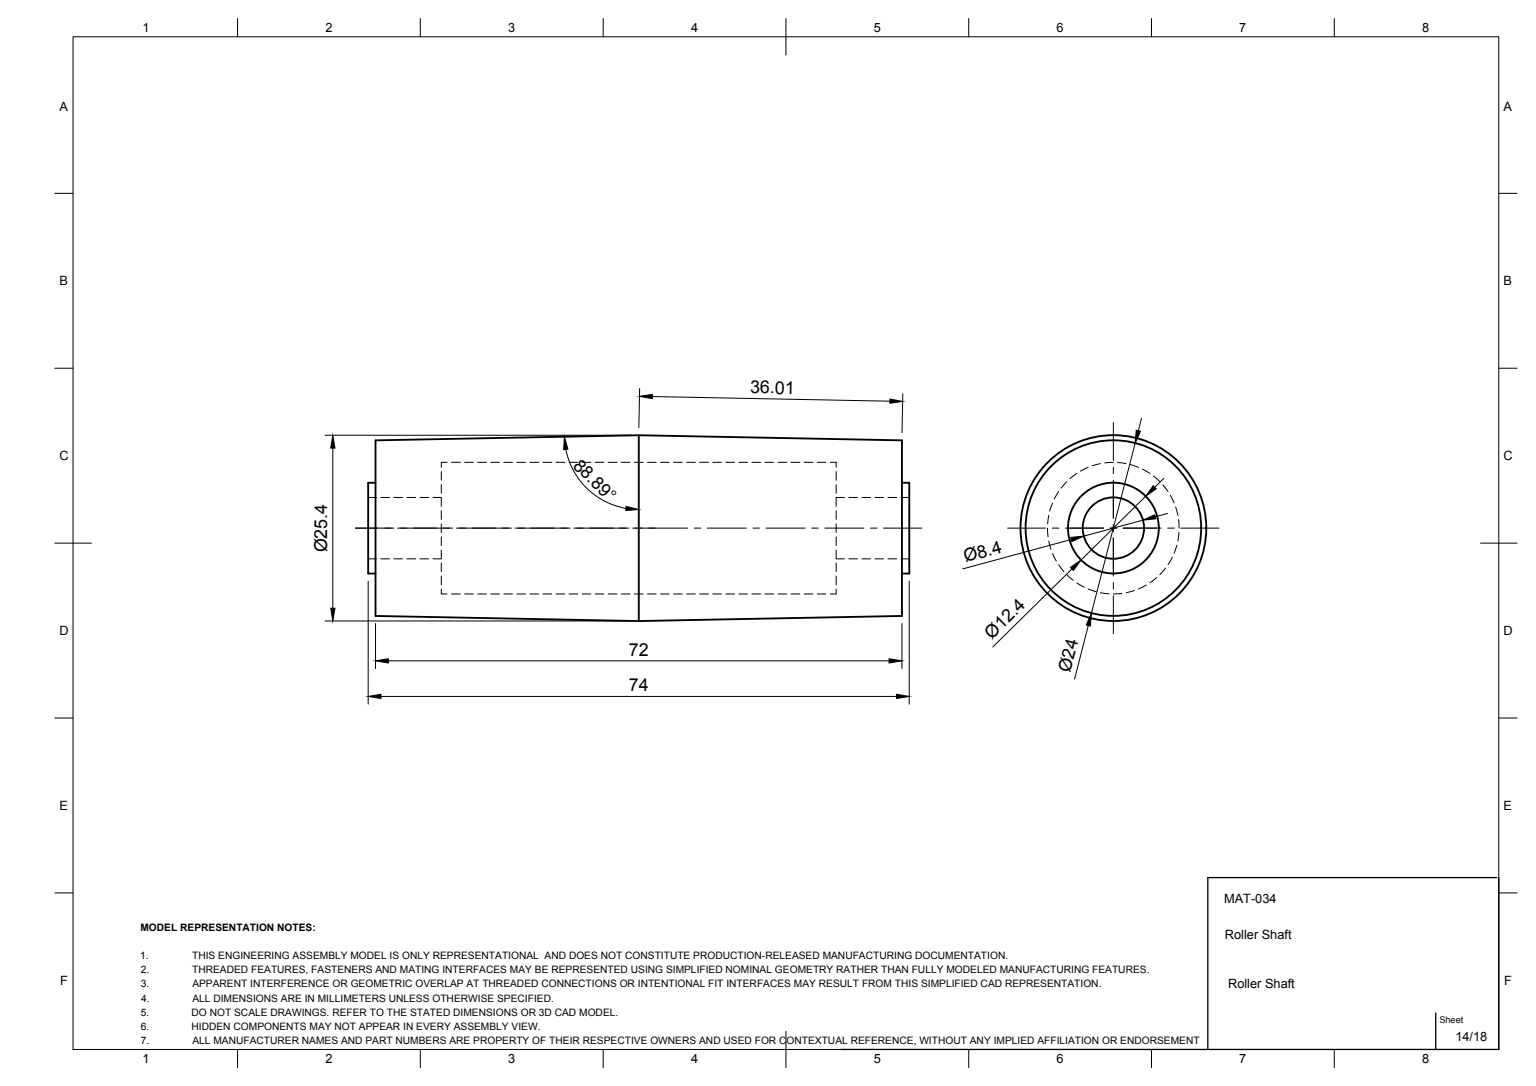
ISO-10303-21;
HEADER;
/* Generated by software containing ST-Developer
 * from STEP Tools, Inc. (www.steptools.com) 
 */

FILE_DESCRIPTION(
/* description */ ('STEP AP214'),
/* implementation_level */ '2;1');

FILE_NAME(
/* name */ 'Roller Shaft.step',
/* time_stamp */ '2026-11-14T09:24:36-08:00',
/* author */ (''),
/* organization */ (''),
/* preprocessor_version */ 'ST-DEVELOPER v20.2',
/* originating_system */ 'Autodesk Translation Framework v15.17.0.0',
/* authorisation */ '');

FILE_SCHEMA (('AUTOMOTIVE_DESIGN { 1 0 10303 214 3 1 1 }'));
ENDSEC;

DATA;
#10=MECHANICAL_DESIGN_GEOMETRIC_PRESENTATION_REPRESENTATION('',(#217),#18867);
#130=CONICAL_SURFACE('',#12139,12.7,0.0194419944400805);
#131=CONICAL_SURFACE('',#12143,12.7,0.0194419944400803);
#185=SHAPE_REPRESENTATION_RELATIONSHIP('SRR','None',#18949,#201);
#201=ADVANCED_BREP_SHAPE_REPRESENTATION('',(#241),#18865);
#217=STYLED_ITEM('',(#19027),#241);
#241=MANIFOLD_SOLID_BREP('Body1',#10972);
#367=FACE_BOUND('',#1981,.T.);
#368=FACE_BOUND('',#1983,.T.);
#369=FACE_BOUND('',#1985,.T.);
#370=FACE_BOUND('',#1987,.T.);
#371=FACE_BOUND('',#1989,.T.);
#372=FACE_BOUND('',#1991,.T.);
#711=PLANE('',#12157);
#712=PLANE('',#12158);
#713=PLANE('',#12159);
#714=PLANE('',#12160);
#715=PLANE('',#12161);
#716=PLANE('',#12162);
#1261=FACE_OUTER_BOUND('',#1973,.T.);
#1262=FACE_OUTER_BOUND('',#1974,.T.);
#1263=FACE_OUTER_BOUND('',#1975,.T.);
#1264=FACE_OUTER_BOUND('',#1976,.T.);
#1265=FACE_OUTER_BOUND('',#1977,.T.);
#1266=FACE_OUTER_BOUND('',#1978,.T.);
#1267=FACE_OUTER_BOUND('',#1979,.T.);
#1268=FACE_OUTER_BOUND('',#1980,.T.);
#1269=FACE_OUTER_BOUND('',#1982,.T.);
#1270=FACE_OUTER_BOUND('',#1984,.T.);
#1271=FACE_OUTER_BOUND('',#1986,.T.);
#1272=FACE_OUTER_BOUND('',#1988,.T.);
#1273=FACE_OUTER_BOUND('',#1990,.T.);
#1973=EDGE_LOOP('',(#9936,#9937,#9938,#9939));
#1974=EDGE_LOOP('',(#9940,#9941,#9942,#9943,#9944));
#1975=EDGE_LOOP('',(#9945,#9946,#9947,#9948,#9949));
#1976=EDGE_LOOP('',(#9950,#9951,#9952,#9953));
#1977=EDGE_LOOP('',(#9954,#9955,#9956,#9957));
#1978=EDGE_LOOP('',(#9958,#9959,#9960,#9961));
#1979=EDGE_LOOP('',(#9962,#9963,#9964,#9965));
#1980=EDGE_LOOP('',(#9966));
#1981=EDGE_LOOP('',(#9967));
#1982=EDGE_LOOP('',(#9968));
#1983=EDGE_LOOP('',(#9969));
#1984=EDGE_LOOP('',(#9970));
#1985=EDGE_LOOP('',(#9971));
#1986=EDGE_LOOP('',(#9972));
#1987=EDGE_LOOP('',(#9973));
#1988=EDGE_LOOP('',(#9974));
#1989=EDGE_LOOP('',(#9975));
#1990=EDGE_LOOP('',(#9976));
#1991=EDGE_LOOP('',(#9977));
#3032=LINE('',#18565,#4046);
#3033=LINE('',#18573,#4047);
#3034=LINE('',#18577,#4048);
#3035=LINE('',#18583,#4049);
#3036=LINE('',#18589,#4050);
#3037=LINE('',#18595,#4051);
#3038=LINE('',#18601,#4052);
#4046=VECTOR('',#15246,9.);
#4047=VECTOR('',#15255,12.7);
#4048=VECTOR('',#15260,12.7);
#4049=VECTOR('',#15267,6.2);
#4050=VECTOR('',#15274,6.2);
#4051=VECTOR('',#15281,4.2);
#4052=VECTOR('',#15288,4.2);
#4496=CIRCLE('',#12137,9.);
#4497=CIRCLE('',#12138,9.);
#4498=CIRCLE('',#12140,12.7);
#4499=CIRCLE('',#12141,12.7);
#4500=CIRCLE('',#12142,12.);
#4501=CIRCLE('',#12144,12.);
#4502=CIRCLE('',#12146,6.2);
#4503=CIRCLE('',#12147,6.2);
#4504=CIRCLE('',#12149,6.2);
#4505=CIRCLE('',#12150,6.2);
#4506=CIRCLE('',#12152,4.2);
#4507=CIRCLE('',#12153,4.2);
#4508=CIRCLE('',#12155,4.2);
#4509=CIRCLE('',#12156,4.2);
#5512=VERTEX_POINT('',#18562);
#5513=VERTEX_POINT('',#18564);
#5514=VERTEX_POINT('',#18568);
#5515=VERTEX_POINT('',#18569);
#5516=VERTEX_POINT('',#18572);
#5517=VERTEX_POINT('',#18576);
#5518=VERTEX_POINT('',#18580);
#5519=VERTEX_POINT('',#18582);
#5520=VERTEX_POINT('',#18586);
#5521=VERTEX_POINT('',#18588);
#5522=VERTEX_POINT('',#18592);
#5523=VERTEX_POINT('',#18594);
#5524=VERTEX_POINT('',#18598);
#5525=VERTEX_POINT('',#18600);
#7001=EDGE_CURVE('',#5512,#5512,#4496,.T.);
#7002=EDGE_CURVE('',#5512,#5513,#3032,.T.);
#7003=EDGE_CURVE('',#5513,#5513,#4497,.T.);
#7004=EDGE_CURVE('',#5514,#5515,#4498,.T.);
#7005=EDGE_CURVE('',#5515,#5514,#4499,.T.);
#7006=EDGE_CURVE('',#5515,#5516,#3033,.T.);
#7007=EDGE_CURVE('',#5516,#5516,#4500,.T.);
#7008=EDGE_CURVE('',#5514,#5517,#3034,.T.);
#7009=EDGE_CURVE('',#5517,#5517,#4501,.T.);
#7010=EDGE_CURVE('',#5518,#5518,#4502,.T.);
#7011=EDGE_CURVE('',#5518,#5519,#3035,.T.);
#7012=EDGE_CURVE('',#5519,#5519,#4503,.T.);
#7013=EDGE_CURVE('',#5520,#5520,#4504,.T.);
#7014=EDGE_CURVE('',#5520,#5521,#3036,.T.);
#7015=EDGE_CURVE('',#5521,#5521,#4505,.T.);
#7016=EDGE_CURVE('',#5522,#5522,#4506,.T.);
#7017=EDGE_CURVE('',#5522,#5523,#3037,.T.);
#7018=EDGE_CURVE('',#5523,#5523,#4507,.T.);
#7019=EDGE_CURVE('',#5524,#5524,#4508,.T.);
#7020=EDGE_CURVE('',#5524,#5525,#3038,.T.);
#7021=EDGE_CURVE('',#5525,#5525,#4509,.T.);
#9936=ORIENTED_EDGE('',*,*,#7001,.F.);
#9937=ORIENTED_EDGE('',*,*,#7002,.T.);
#9938=ORIENTED_EDGE('',*,*,#7003,.T.);
#9939=ORIENTED_EDGE('',*,*,#7002,.F.);
#9940=ORIENTED_EDGE('',*,*,#7004,.F.);
#9941=ORIENTED_EDGE('',*,*,#7005,.F.);
#9942=ORIENTED_EDGE('',*,*,#7006,.T.);
#9943=ORIENTED_EDGE('',*,*,#7007,.T.);
#9944=ORIENTED_EDGE('',*,*,#7006,.F.);
#9945=ORIENTED_EDGE('',*,*,#7004,.T.);
#9946=ORIENTED_EDGE('',*,*,#7005,.T.);
#9947=ORIENTED_EDGE('',*,*,#7008,.T.);
#9948=ORIENTED_EDGE('',*,*,#7009,.F.);
#9949=ORIENTED_EDGE('',*,*,#7008,.F.);
#9950=ORIENTED_EDGE('',*,*,#7010,.F.);
#9951=ORIENTED_EDGE('',*,*,#7011,.T.);
#9952=ORIENTED_EDGE('',*,*,#7012,.T.);
#9953=ORIENTED_EDGE('',*,*,#7011,.F.);
#9954=ORIENTED_EDGE('',*,*,#7013,.T.);
#9955=ORIENTED_EDGE('',*,*,#7014,.T.);
#9956=ORIENTED_EDGE('',*,*,#7015,.F.);
#9957=ORIENTED_EDGE('',*,*,#7014,.F.);
#9958=ORIENTED_EDGE('',*,*,#7016,.T.);
#9959=ORIENTED_EDGE('',*,*,#7017,.T.);
#9960=ORIENTED_EDGE('',*,*,#7018,.F.);
#9961=ORIENTED_EDGE('',*,*,#7017,.F.);
#9962=ORIENTED_EDGE('',*,*,#7019,.T.);
#9963=ORIENTED_EDGE('',*,*,#7020,.T.);
#9964=ORIENTED_EDGE('',*,*,#7021,.T.);
#9965=ORIENTED_EDGE('',*,*,#7020,.F.);
#9966=ORIENTED_EDGE('',*,*,#7007,.F.);
#9967=ORIENTED_EDGE('',*,*,#7010,.T.);
#9968=ORIENTED_EDGE('',*,*,#7009,.T.);
#9969=ORIENTED_EDGE('',*,*,#7013,.F.);
#9970=ORIENTED_EDGE('',*,*,#7015,.T.);
#9971=ORIENTED_EDGE('',*,*,#7019,.F.);
#9972=ORIENTED_EDGE('',*,*,#7012,.F.);
#9973=ORIENTED_EDGE('',*,*,#7018,.T.);
#9974=ORIENTED_EDGE('',*,*,#7003,.F.);
#9975=ORIENTED_EDGE('',*,*,#7021,.F.);
#9976=ORIENTED_EDGE('',*,*,#7001,.T.);
#9977=ORIENTED_EDGE('',*,*,#7016,.F.);
#10345=CYLINDRICAL_SURFACE('',#12136,9.);
#10346=CYLINDRICAL_SURFACE('',#12145,6.2);
#10347=CYLINDRICAL_SURFACE('',#12148,6.2);
#10348=CYLINDRICAL_SURFACE('',#12151,4.2);
#10349=CYLINDRICAL_SURFACE('',#12154,4.2);
#10898=ADVANCED_FACE('',(#1261),#10345,.F.);
#10899=ADVANCED_FACE('',(#1262),#130,.T.);
#10900=ADVANCED_FACE('',(#1263),#131,.T.);
#10901=ADVANCED_FACE('',(#1264),#10346,.T.);
#10902=ADVANCED_FACE('',(#1265),#10347,.T.);
#10903=ADVANCED_FACE('',(#1266),#10348,.F.);
#10904=ADVANCED_FACE('',(#1267),#10349,.F.);
#10905=ADVANCED_FACE('',(#1268,#367),#711,.F.);
#10906=ADVANCED_FACE('',(#1269,#368),#712,.T.);
#10907=ADVANCED_FACE('',(#1270,#369),#713,.T.);
#10908=ADVANCED_FACE('',(#1271,#370),#714,.T.);
#10909=ADVANCED_FACE('',(#1272,#371),#715,.T.);
#10910=ADVANCED_FACE('',(#1273,#372),#716,.T.);
#10972=CLOSED_SHELL('',(#10898,#10899,#10900,#10901,#10902,#10903,#10904,
#10905,#10906,#10907,#10908,#10909,#10910));
#12135=AXIS2_PLACEMENT_3D('',#18560,#15240,#15241);
#12136=AXIS2_PLACEMENT_3D('',#18561,#15242,#15243);
#12137=AXIS2_PLACEMENT_3D('',#18563,#15244,#15245);
#12138=AXIS2_PLACEMENT_3D('',#18566,#15247,#15248);
#12139=AXIS2_PLACEMENT_3D('',#18567,#15249,#15250);
#12140=AXIS2_PLACEMENT_3D('',#18570,#15251,#15252);
#12141=AXIS2_PLACEMENT_3D('',#18571,#15253,#15254);
#12142=AXIS2_PLACEMENT_3D('',#18574,#15256,#15257);
#12143=AXIS2_PLACEMENT_3D('',#18575,#15258,#15259);
#12144=AXIS2_PLACEMENT_3D('',#18578,#15261,#15262);
#12145=AXIS2_PLACEMENT_3D('',#18579,#15263,#15264);
#12146=AXIS2_PLACEMENT_3D('',#18581,#15265,#15266);
#12147=AXIS2_PLACEMENT_3D('',#18584,#15268,#15269);
#12148=AXIS2_PLACEMENT_3D('',#18585,#15270,#15271);
#12149=AXIS2_PLACEMENT_3D('',#18587,#15272,#15273);
#12150=AXIS2_PLACEMENT_3D('',#18590,#15275,#15276);
#12151=AXIS2_PLACEMENT_3D('',#18591,#15277,#15278);
#12152=AXIS2_PLACEMENT_3D('',#18593,#15279,#15280);
#12153=AXIS2_PLACEMENT_3D('',#18596,#15282,#15283);
#12154=AXIS2_PLACEMENT_3D('',#18597,#15284,#15285);
#12155=AXIS2_PLACEMENT_3D('',#18599,#15286,#15287);
#12156=AXIS2_PLACEMENT_3D('',#18602,#15289,#15290);
#12157=AXIS2_PLACEMENT_3D('',#18603,#15291,#15292);
#12158=AXIS2_PLACEMENT_3D('',#18604,#15293,#15294);
#12159=AXIS2_PLACEMENT_3D('',#18605,#15295,#15296);
#12160=AXIS2_PLACEMENT_3D('',#18606,#15297,#15298);
#12161=AXIS2_PLACEMENT_3D('',#18607,#15299,#15300);
#12162=AXIS2_PLACEMENT_3D('',#18608,#15301,#15302);
#15240=DIRECTION('axis',(0.,0.,1.));
#15241=DIRECTION('refdir',(1.,0.,0.));
#15242=DIRECTION('center_axis',(0.,0.,1.));
#15243=DIRECTION('ref_axis',(1.,0.,0.));
#15244=DIRECTION('center_axis',(0.,0.,1.));
#15245=DIRECTION('ref_axis',(1.,0.,0.));
#15246=DIRECTION('',(0.,0.,1.));
#15247=DIRECTION('center_axis',(0.,0.,1.));
#15248=DIRECTION('ref_axis',(1.,0.,0.));
#15249=DIRECTION('center_axis',(0.,0.,1.));
#15250=DIRECTION('ref_axis',(1.,0.,0.));
#15251=DIRECTION('center_axis',(0.,0.,1.));
#15252=DIRECTION('ref_axis',(1.,0.,0.));
#15253=DIRECTION('center_axis',(0.,0.,1.));
#15254=DIRECTION('ref_axis',(1.,0.,0.));
#15255=DIRECTION('',(0.0194407696462631,2.38080763202572E-18,-0.999811010379242));
#15256=DIRECTION('center_axis',(0.,0.,1.));
#15257=DIRECTION('ref_axis',(1.,0.,0.));
#15258=DIRECTION('center_axis',(0.,0.,-1.));
#15259=DIRECTION('ref_axis',(-1.,0.,0.));
#15260=DIRECTION('',(-0.0194407696462629,2.38080763202569E-18,0.999811010379242));
#15261=DIRECTION('center_axis',(0.,0.,1.));
#15262=DIRECTION('ref_axis',(1.,0.,0.));
#15263=DIRECTION('center_axis',(0.,0.,1.));
#15264=DIRECTION('ref_axis',(1.,0.,0.));
#15265=DIRECTION('center_axis',(0.,0.,1.));
#15266=DIRECTION('ref_axis',(1.,0.,0.));
#15267=DIRECTION('',(0.,0.,-1.));
#15268=DIRECTION('center_axis',(0.,0.,1.));
#15269=DIRECTION('ref_axis',(1.,0.,0.));
#15270=DIRECTION('center_axis',(0.,0.,-1.));
#15271=DIRECTION('ref_axis',(-1.,0.,0.));
#15272=DIRECTION('center_axis',(0.,0.,1.));
#15273=DIRECTION('ref_axis',(1.,0.,0.));
#15274=DIRECTION('',(0.,0.,1.));
#15275=DIRECTION('center_axis',(0.,0.,1.));
#15276=DIRECTION('ref_axis',(1.,0.,0.));
#15277=DIRECTION('center_axis',(0.,0.,-1.));
#15278=DIRECTION('ref_axis',(-1.,0.,0.));
#15279=DIRECTION('center_axis',(0.,0.,1.));
#15280=DIRECTION('ref_axis',(1.,0.,0.));
#15281=DIRECTION('',(0.,0.,-1.));
#15282=DIRECTION('center_axis',(0.,0.,1.));
#15283=DIRECTION('ref_axis',(1.,0.,0.));
#15284=DIRECTION('center_axis',(0.,0.,-1.));
#15285=DIRECTION('ref_axis',(-1.,0.,0.));
#15286=DIRECTION('center_axis',(0.,0.,1.));
#15287=DIRECTION('ref_axis',(1.,0.,0.));
#15288=DIRECTION('',(0.,0.,-1.));
#15289=DIRECTION('center_axis',(0.,0.,-1.));
#15290=DIRECTION('ref_axis',(-1.,0.,0.));
#15291=DIRECTION('center_axis',(0.,0.,1.));
#15292=DIRECTION('ref_axis',(1.,0.,0.));
#15293=DIRECTION('center_axis',(0.,0.,1.));
#15294=DIRECTION('ref_axis',(1.,0.,0.));
#15295=DIRECTION('center_axis',(0.,0.,1.));
#15296=DIRECTION('ref_axis',(1.,0.,0.));
#15297=DIRECTION('center_axis',(0.,0.,-1.));
#15298=DIRECTION('ref_axis',(1.,0.,0.));
#15299=DIRECTION('center_axis',(0.,0.,-1.));
#15300=DIRECTION('ref_axis',(-1.,0.,0.));
#15301=DIRECTION('center_axis',(0.,0.,1.));
#15302=DIRECTION('ref_axis',(1.,0.,0.));
#18560=CARTESIAN_POINT('',(0.,0.,0.));
#18561=CARTESIAN_POINT('Origin',(0.,0.,37.));
#18562=CARTESIAN_POINT('',(-9.,-1.10218211923262E-15,-27.));
#18563=CARTESIAN_POINT('Origin',(0.,0.,-27.));
#18564=CARTESIAN_POINT('',(-9.,-1.10218211923262E-15,27.));
#18565=CARTESIAN_POINT('',(-9.,-1.10218211923262E-15,37.));
#18566=CARTESIAN_POINT('Origin',(0.,0.,27.));
#18567=CARTESIAN_POINT('Origin',(0.,0.,-1.45716771982052E-13));
#18568=CARTESIAN_POINT('',(12.7,1.55530143491714E-15,-1.45716771982052E-13));
#18569=CARTESIAN_POINT('',(-12.7,-1.55530143491714E-15,-1.45716771982052E-13));
#18570=CARTESIAN_POINT('Origin',(0.,0.,-1.45716771982052E-13));
#18571=CARTESIAN_POINT('Origin',(0.,0.,-1.45716771982052E-13));
#18572=CARTESIAN_POINT('',(-12.,-1.46957615897682E-15,-36.));
#18573=CARTESIAN_POINT('',(-12.7,-1.55530143491714E-15,-1.45716771982052E-13));
#18574=CARTESIAN_POINT('Origin',(0.,0.,-36.));
#18575=CARTESIAN_POINT('Origin',(0.,0.,-1.45716771982052E-13));
#18576=CARTESIAN_POINT('',(12.,-1.46957615897682E-15,36.));
#18577=CARTESIAN_POINT('',(12.7,-1.55530143491714E-15,-1.45716771982052E-13));
#18578=CARTESIAN_POINT('Origin',(0.,0.,36.));
#18579=CARTESIAN_POINT('Origin',(0.,0.,-37.));
#18580=CARTESIAN_POINT('',(-6.2,-7.59281015471359E-16,-36.));
#18581=CARTESIAN_POINT('Origin',(0.,0.,-36.));
#18582=CARTESIAN_POINT('',(-6.2,-7.59281015471359E-16,-37.));
#18583=CARTESIAN_POINT('',(-6.2,-7.59281015471359E-16,-37.));
#18584=CARTESIAN_POINT('Origin',(0.,0.,-37.));
#18585=CARTESIAN_POINT('Origin',(0.,0.,37.));
#18586=CARTESIAN_POINT('',(6.2,-7.59281015471359E-16,36.));
#18587=CARTESIAN_POINT('Origin',(0.,0.,36.));
#18588=CARTESIAN_POINT('',(6.2,-7.59281015471359E-16,37.));
#18589=CARTESIAN_POINT('',(6.2,-7.59281015471359E-16,37.));
#18590=CARTESIAN_POINT('Origin',(0.,0.,37.));
#18591=CARTESIAN_POINT('Origin',(0.,0.,36.));
#18592=CARTESIAN_POINT('',(4.2,-5.14351655641888E-16,-27.));
#18593=CARTESIAN_POINT('Origin',(0.,0.,-27.));
#18594=CARTESIAN_POINT('',(4.2,-5.14351655641888E-16,-37.));
#18595=CARTESIAN_POINT('',(4.2,-5.14351655641888E-16,36.));
#18596=CARTESIAN_POINT('Origin',(0.,0.,-37.));
#18597=CARTESIAN_POINT('Origin',(0.,0.,36.));
#18598=CARTESIAN_POINT('',(4.2,-5.14351655641888E-16,37.));
#18599=CARTESIAN_POINT('Origin',(0.,0.,37.));
#18600=CARTESIAN_POINT('',(4.2,-5.14351655641888E-16,27.));
#18601=CARTESIAN_POINT('',(4.2,-5.14351655641888E-16,36.));
#18602=CARTESIAN_POINT('Origin',(0.,0.,27.));
#18603=CARTESIAN_POINT('Origin',(0.,0.,-36.));
#18604=CARTESIAN_POINT('Origin',(0.,0.,36.));
#18605=CARTESIAN_POINT('Origin',(0.,0.,37.));
#18606=CARTESIAN_POINT('Origin',(0.,0.,-37.));
#18607=CARTESIAN_POINT('Origin',(0.,0.,27.));
#18608=CARTESIAN_POINT('Origin',(0.,0.,-27.));
#18847=UNCERTAINTY_MEASURE_WITH_UNIT(LENGTH_MEASURE(0.01),#18868,
'DISTANCE_ACCURACY_VALUE',
'Maximum model space distance between geometric entities at asserted c
onnectivities');
#18849=UNCERTAINTY_MEASURE_WITH_UNIT(LENGTH_MEASURE(0.01),#18868,
'DISTANCE_ACCURACY_VALUE',
'Maximum model space distance between geometric entities at asserted c
onnectivities');
#18865=(
GEOMETRIC_REPRESENTATION_CONTEXT(3)
GLOBAL_UNCERTAINTY_ASSIGNED_CONTEXT((#18847))
GLOBAL_UNIT_ASSIGNED_CONTEXT((#18868,#18870,#18871))
REPRESENTATION_CONTEXT('','3D')
);
#18867=(
GEOMETRIC_REPRESENTATION_CONTEXT(3)
GLOBAL_UNCERTAINTY_ASSIGNED_CONTEXT((#18849))
GLOBAL_UNIT_ASSIGNED_CONTEXT((#18868,#18870,#18871))
REPRESENTATION_CONTEXT('','3D')
);
#18868=(
LENGTH_UNIT()
NAMED_UNIT(*)
SI_UNIT(.MILLI.,.METRE.)
);
#18870=(
NAMED_UNIT(*)
PLANE_ANGLE_UNIT()
SI_UNIT($,.RADIAN.)
);
#18871=(
NAMED_UNIT(*)
SI_UNIT($,.STERADIAN.)
SOLID_ANGLE_UNIT()
);
#18887=SHAPE_DEFINITION_REPRESENTATION(#18904,#18949);
#18904=PRODUCT_DEFINITION_SHAPE('',$,#18967);
#18949=SHAPE_REPRESENTATION('',(#12135),#18865);
#18951=PRODUCT_DEFINITION_CONTEXT('part definition',#19004,'design');
#18967=PRODUCT_DEFINITION('Roller Shaft','Roller Shaft',#18984,#18951);
#18984=PRODUCT_DEFINITION_FORMATION('',$,#19021);
#19004=APPLICATION_CONTEXT(
'Core Data for Automotive Mechanical Design Process');
#19005=PRODUCT_CONTEXT('part definition',#19004,'mechanical');
#19021=PRODUCT('Roller Shaft','Roller Shaft',$,(#19005));
#19027=PRESENTATION_STYLE_ASSIGNMENT((#19033));
#19033=SURFACE_STYLE_USAGE(.BOTH.,#19039);
#19039=SURFACE_SIDE_STYLE('',(#19045));
#19045=SURFACE_STYLE_FILL_AREA(#19051);
#19051=FILL_AREA_STYLE('Opaque(122,133,145)',(#19057));
#19057=FILL_AREA_STYLE_COLOUR('Opaque(122,133,145)',#19063);
#19063=COLOUR_RGB('Opaque(122,133,145)',0.47843137254902,0.52156862745098,
0.568627450980392);
ENDSEC;
END-ISO-10303-21;
